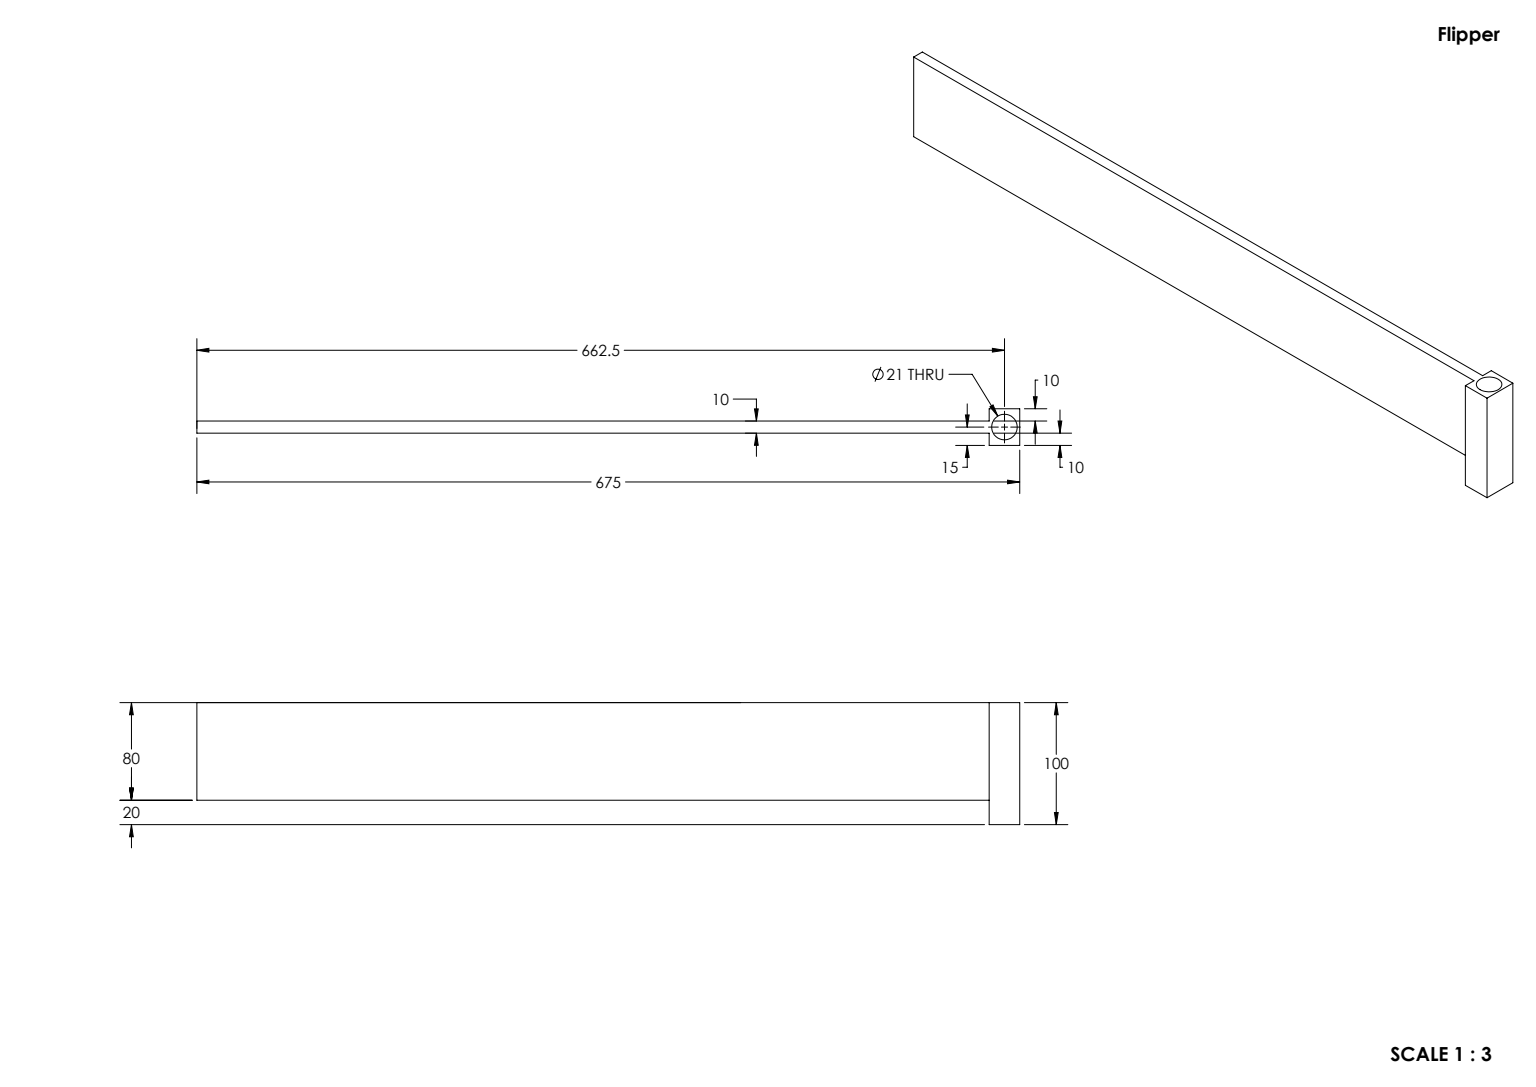
ISO-10303-21;
HEADER;
FILE_DESCRIPTION (('STEP AP214'),
    '1' );
FILE_NAME ('Flipper.step',
    '2026-10-24T15:53:57',
    ( '' ),
    ( '' ),
    'SwSTEP 2.0',
    'SolidWorks 2025',
    '' );
FILE_SCHEMA (( 'AUTOMOTIVE_DESIGN' ));
ENDSEC;

DATA;
#20=MANIFOLD_SOLID_BREP ( 'Cut-Extrude1', #1796 ) ;
#27=EDGE_CURVE ( 'NONE', #6851, #3192, #686, .T. ) ;
#51=PLANE ( 'NONE',  #3089 ) ;
#86=CARTESIAN_POINT ( 'NONE',  ( 5.000000000000115463, -14.99999999999990230, 79.99999999999995737 ) ) ;
#119=CARTESIAN_POINT ( 'NONE',  ( 5.000000000000115463, -14.99999999999990230, 79.99999999999995737 ) ) ;
#159=ORIENTED_EDGE ( 'NONE', *, *, #1330, .T. ) ;
#182=CARTESIAN_POINT ( 'NONE',  ( 10.00000000000012079, -29.14213562373080180, 0.000000000000000000 ) ) ;
#214=ORIENTED_EDGE ( 'NONE', *, *, #1634, .F. ) ;
#218=VERTEX_POINT ( 'NONE', #2995 ) ;
#231=CARTESIAN_POINT ( 'NONE',  ( 5.000000000000115463, -14.99999999999990230, -20.00100000000004741 ) ) ;
#242=VECTOR ( 'NONE', #7821, 1000.000000000000000 ) ;
#252=DIRECTION ( 'NONE',  ( -7.420547859534711256E-34, 1.000000000000000000, 1.224646799147352961E-16 ) ) ;
#253=DIRECTION ( 'NONE',  ( -7.703719777548943412E-34, 0.000000000000000000, 1.000000000000000000 ) ) ;
#256=DIRECTION ( 'NONE',  ( -7.420547859534711256E-34, 1.000000000000000000, 1.224646799147352961E-16 ) ) ;
#261=DIRECTION ( 'NONE',  ( 0.000000000000000000, -1.000000000000000000, -1.224646799147352714E-16 ) ) ;
#262=ADVANCED_FACE ( 'NONE', ( #7614 ), #6970, .T. ) ;
#284=ORIENTED_EDGE ( 'NONE', *, *, #3202, .F. ) ;
#302=ORIENTED_EDGE ( 'NONE', *, *, #1070, .T. ) ;
#303=VERTEX_POINT ( 'NONE', #1894 ) ;
#313=CARTESIAN_POINT ( 'NONE',  ( -9.999999999999884537, -14.99999999999990052, -20.00000000000001776 ) ) ;
#318=ADVANCED_FACE ( 'NONE', ( #509 ), #5075, .F. ) ;
#332=ADVANCED_FACE ( 'NONE', ( #3201 ), #4425, .F. ) ;
#340=CARTESIAN_POINT ( 'NONE',  ( 5.000000000000115463, -14.99999999999990230, -20.00000000000001776 ) ) ;
#359=VECTOR ( 'NONE', #6067, 1000.000000000000000 ) ;
#368=CYLINDRICAL_SURFACE ( 'NONE', #7232, 10.49999999999999645 ) ;
#421=CARTESIAN_POINT ( 'NONE',  ( 9.999999999999896971, 0.000000000000000000, 0.000000000000000000 ) ) ;
#441=CARTESIAN_POINT ( 'NONE',  ( 10.00000000000000888, -650.0000000000002274, 79.99999999999995737 ) ) ;
#458=CARTESIAN_POINT ( 'NONE',  ( 10.00000000000000888, -0.8578643762688908936, 0.000000000000000000 ) ) ;
#479=AXIS2_PLACEMENT_3D ( 'NONE', #3533, #253, #2914 ) ;
#499=DIRECTION ( 'NONE',  ( -7.703719777548943412E-34, 0.000000000000000000, 1.000000000000000000 ) ) ;
#509=FACE_OUTER_BOUND ( 'NONE', #3864, .T. ) ;
#519=ORIENTED_EDGE ( 'NONE', *, *, #7936, .T. ) ;
#530=VERTEX_POINT ( 'NONE', #3474 ) ;
#550=LINE ( 'NONE', #5350, #242 ) ;
#558=EDGE_CURVE ( 'NONE', #4476, #8418, #2901, .T. ) ;
#565=LINE ( 'NONE', #5367, #5443 ) ;
#581=CIRCLE ( 'NONE', #5462, 15.00000000000000355 ) ;
#622=CARTESIAN_POINT ( 'NONE',  ( 5.000000000000004441, 0.000000000000000000, 0.000000000000000000 ) ) ;
#624=ORIENTED_EDGE ( 'NONE', *, *, #8030, .T. ) ;
#627=ORIENTED_EDGE ( 'NONE', *, *, #1962, .T. ) ;
#630=ORIENTED_EDGE ( 'NONE', *, *, #1968, .T. ) ;
#686=LINE ( 'NONE', #6066, #6271 ) ;
#718=ORIENTED_EDGE ( 'NONE', *, *, #558, .T. ) ;
#731=LINE ( 'NONE', #3391, #359 ) ;
#774=( LENGTH_UNIT ( ) NAMED_UNIT ( * ) SI_UNIT ( .MILLI., .METRE. ) );
#800=DIRECTION ( 'NONE',  ( 1.000000000000000000, 0.000000000000000000, 0.000000000000000000 ) ) ;
#826=CIRCLE ( 'NONE', #1930, 10.49999999999999645 ) ;
#832=ORIENTED_EDGE ( 'NONE', *, *, #6918, .T. ) ;
#843=DIRECTION ( 'NONE',  ( 4.622231866529366732E-33, -1.224646799147352961E-16, 1.000000000000000000 ) ) ;
#846=EDGE_CURVE ( 'NONE', #4479, #218, #4939, .T. ) ;
#860=( NAMED_UNIT ( * ) PLANE_ANGLE_UNIT ( ) SI_UNIT ( $, .RADIAN. ) );
#883=VECTOR ( 'NONE', #4658, 1000.000000000000000 ) ;
#898=FACE_OUTER_BOUND ( 'NONE', #6189, .T. ) ;
#899=EDGE_CURVE ( 'NONE', #7534, #6851, #5991, .T. ) ;
#942=CARTESIAN_POINT ( 'NONE',  ( 10.00000000000000888, -650.0000000000002274, 79.99999999999995737 ) ) ;
#959=CIRCLE ( 'NONE', #5553, 15.00000000000000355 ) ;
#961=CARTESIAN_POINT ( 'NONE',  ( 0.000000000000000000, 0.000000000000000000, 0.000000000000000000 ) ) ;
#968=DIRECTION ( 'NONE',  ( -7.703719777548943412E-34, 0.000000000000000000, 1.000000000000000000 ) ) ;
#992=ORIENTED_EDGE ( 'NONE', *, *, #3308, .F. ) ;
#1006=EDGE_LOOP ( 'NONE', ( #2429, #302, #624, #3207, #7185, #3525, #718, #4684 ) ) ;
#1061=CARTESIAN_POINT ( 'NONE',  ( 15.50000000000011191, -14.99999999999990230, 79.99999999999995737 ) ) ;
#1066=FACE_BOUND ( 'NONE', #7624, .T. ) ;
#1070=EDGE_CURVE ( 'NONE', #8094, #5152, #5051, .T. ) ;
#1087=CARTESIAN_POINT ( 'NONE',  ( 5.000000000000115463, -14.99999999999990230, 0.000000000000000000 ) ) ;
#1127=DIRECTION ( 'NONE',  ( 2.842664852890546338E-35, -1.000000000000000000, 0.000000000000000000 ) ) ;
#1132=UNCERTAINTY_MEASURE_WITH_UNIT (LENGTH_MEASURE( 1.000000000000000082E-05 ), #1546, 'distance_accuracy_value', 'NONE');
#1140=AXIS2_PLACEMENT_3D ( 'NONE', #6510, #5843, #8469 ) ;
#1162=ORIENTED_EDGE ( 'NONE', *, *, #899, .F. ) ;
#1170=ADVANCED_FACE ( 'NONE', ( #3127 ), #3214, .F. ) ;
#1253=VECTOR ( 'NONE', #5699, 1000.000000000000000 ) ;
#1255=FACE_OUTER_BOUND ( 'NONE', #4456, .T. ) ;
#1308=CARTESIAN_POINT ( 'NONE',  ( -2.220446049250313081E-13, -650.0000000000000000, -1.110223024625156540E-13 ) ) ;
#1330=EDGE_CURVE ( 'NONE', #530, #3192, #731, .T. ) ;
#1337=VERTEX_POINT ( 'NONE', #8226 ) ;
#1352=CARTESIAN_POINT ( 'NONE',  ( 20.00000000000011369, -14.99999999999990230, 79.99999999999995737 ) ) ;
#1359=ORIENTED_EDGE ( 'NONE', *, *, #3242, .T. ) ;
#1364=CARTESIAN_POINT ( 'NONE',  ( 5.000000000000115463, -14.99999999999990230, 79.99999999999995737 ) ) ;
#1388=LINE ( 'NONE', #5356, #4852 ) ;
#1390=CARTESIAN_POINT ( 'NONE',  ( 15.50000000000011191, -14.99999999999990230, -20.00100000000004741 ) ) ;
#1392=( GEOMETRIC_REPRESENTATION_CONTEXT ( 3 ) GLOBAL_UNCERTAINTY_ASSIGNED_CONTEXT ( ( #7343 ) ) GLOBAL_UNIT_ASSIGNED_CONTEXT ( ( #774, #7439, #8135 ) ) REPRESENTATION_CONTEXT ( 'NONE', 'WORKASPACE' ) );
#1393=DIRECTION ( 'NONE',  ( -1.000000000000000000, 2.842664852890546338E-35, 1.540743955509788340E-33 ) ) ;
#1397=CARTESIAN_POINT ( 'NONE',  ( 5.000000000000115463, -14.99999999999990230, -20.00100000000004741 ) ) ;
#1427=AXIS2_PLACEMENT_3D ( 'NONE', #5540, #6844, #1518 ) ;
#1449=CARTESIAN_POINT ( 'NONE',  ( 9.999999999999896971, 0.000000000000000000, 0.000000000000000000 ) ) ;
#1461=EDGE_CURVE ( 'NONE', #7908, #6954, #5531, .T. ) ;
#1465=DIRECTION ( 'NONE',  ( -1.000000000000000000, 2.842664852890546338E-35, -7.703719777548943412E-34 ) ) ;
#1478=ORIENTED_EDGE ( 'NONE', *, *, #1070, .F. ) ;
#1495=ORIENTED_EDGE ( 'NONE', *, *, #1461, .T. ) ;
#1518=DIRECTION ( 'NONE',  ( 1.000000000000000000, 0.000000000000000000, 0.000000000000000000 ) ) ;
#1546=( LENGTH_UNIT ( ) NAMED_UNIT ( * ) SI_UNIT ( .MILLI., .METRE. ) );
#1549=ORIENTED_EDGE ( 'NONE', *, *, #4424, .T. ) ;
#1552=CARTESIAN_POINT ( 'NONE',  ( 0.000000000000000000, 0.000000000000000000, 0.000000000000000000 ) ) ;
#1582=CARTESIAN_POINT ( 'NONE',  ( 9.999999999999896971, 0.000000000000000000, 79.99999999999995737 ) ) ;
#1584=EDGE_CURVE ( 'NONE', #8094, #2182, #6432, .T. ) ;
#1620=DIRECTION ( 'NONE',  ( -1.000000000000000000, 2.842664852890546338E-35, 1.540743955509788340E-33 ) ) ;
#1634=EDGE_CURVE ( 'NONE', #2098, #1337, #5074, .T. ) ;
#1646=CARTESIAN_POINT ( 'NONE',  ( 5.000000000000115463, -14.99999999999990230, 0.000000000000000000 ) ) ;
#1660=AXIS2_PLACEMENT_3D ( 'NONE', #1364, #4015, #6635 ) ;
#1661=EDGE_CURVE ( 'NONE', #1337, #4479, #4550, .T. ) ;
#1716=VERTEX_POINT ( 'NONE', #3373 ) ;
#1748=VECTOR ( 'NONE', #8434, 1000.000000000000000 ) ;
#1757=ORIENTED_EDGE ( 'NONE', *, *, #1584, .T. ) ;
#1766=ADVANCED_FACE ( 'NONE', ( #6825 ), #2170, .T. ) ;
#1775=CARTESIAN_POINT ( 'NONE',  ( 5.000000000000115463, -14.99999999999990230, -20.00000000000001776 ) ) ;
#1796=CLOSED_SHELL ( 'NONE', ( #5165, #5744, #3088, #4851, #318, #262, #4059, #4277, #1170, #4627, #332, #5630, #1766, #4762, #3103 ) ) ;
#1823=DIRECTION ( 'NONE',  ( 1.000000000000000000, -2.842664852890546338E-35, -1.540743955509788340E-33 ) ) ;
#1835=AXIS2_PLACEMENT_3D ( 'NONE', #1397, #4571, #7970 ) ;
#1838=ORIENTED_EDGE ( 'NONE', *, *, #6705, .F. ) ;
#1894=CARTESIAN_POINT ( 'NONE',  ( 0.000000000000000000, 0.000000000000000000, 79.99999999999995737 ) ) ;
#1908=DIRECTION ( 'NONE',  ( -2.842664852890546338E-35, 1.000000000000000000, -2.189909344815615958E-68 ) ) ;
#1918=CARTESIAN_POINT ( 'NONE',  ( 9.999999999999896971, 0.000000000000000000, 0.000000000000000000 ) ) ;
#1930=AXIS2_PLACEMENT_3D ( 'NONE', #3172, #8488, #2522 ) ;
#1935=EDGE_LOOP ( 'NONE', ( #6404, #7360, #7630 ) ) ;
#1962=EDGE_CURVE ( 'NONE', #2182, #8418, #8061, .T. ) ;
#1968=EDGE_CURVE ( 'NONE', #5323, #2931, #2361, .T. ) ;
#2048=ORIENTED_EDGE ( 'NONE', *, *, #5752, .F. ) ;
#2098=VERTEX_POINT ( 'NONE', #458 ) ;
#2105=AXIS2_PLACEMENT_3D ( 'NONE', #1646, #2967, #261 ) ;
#2128=FACE_OUTER_BOUND ( 'NONE', #4821, .T. ) ;
#2132=EDGE_CURVE ( 'NONE', #8150, #6642, #5440, .T. ) ;
#2157=APPLICATION_CONTEXT ( 'automotive_design' ) ;
#2170=CYLINDRICAL_SURFACE ( 'NONE', #3581, 15.00000000000000355 ) ;
#2178=EDGE_CURVE ( 'NONE', #218, #303, #4541, .T. ) ;
#2182=VERTEX_POINT ( 'NONE', #7938 ) ;
#2248=EDGE_LOOP ( 'NONE', ( #6424, #4523 ) ) ;
#2261=AXIS2_PLACEMENT_3D ( 'NONE', #7188, #5267, #6624 ) ;
#2279=DIRECTION ( 'NONE',  ( 1.000000000000000000, 0.000000000000000000, 0.000000000000000000 ) ) ;
#2306=VECTOR ( 'NONE', #2824, 1000.000000000000000 ) ;
#2357=VECTOR ( 'NONE', #7940, 1000.000000000000000 ) ;
#2361=LINE ( 'NONE', #7639, #2490 ) ;
#2370=CIRCLE ( 'NONE', #4607, 10.49999999999999645 ) ;
#2416=DIRECTION ( 'NONE',  ( 2.842664852890546338E-35, -1.000000000000000000, 0.000000000000000000 ) ) ;
#2429=ORIENTED_EDGE ( 'NONE', *, *, #1584, .F. ) ;
#2440=CARTESIAN_POINT ( 'NONE',  ( 9.999999999999896971, 0.000000000000000000, 79.99999999999995737 ) ) ;
#2442=ORIENTED_EDGE ( 'NONE', *, *, #1634, .T. ) ;
#2470=CARTESIAN_POINT ( 'NONE',  ( 15.50000000000011191, -14.99999999999990230, -20.00000000000001776 ) ) ;
#2477=AXIS2_PLACEMENT_3D ( 'NONE', #1775, #7223, #3788 ) ;
#2490=VECTOR ( 'NONE', #3020, 1000.000000000000000 ) ;
#2522=DIRECTION ( 'NONE',  ( 1.000000000000000000, 0.000000000000000000, 0.000000000000000000 ) ) ;
#2533=CIRCLE ( 'NONE', #1427, 10.49999999999999645 ) ;
#2542=VECTOR ( 'NONE', #4532, 1000.000000000000000 ) ;
#2613=CARTESIAN_POINT ( 'NONE',  ( 10.00000000000000888, -650.0000000000002274, 79.99999999999995737 ) ) ;
#2654=CARTESIAN_POINT ( 'NONE',  ( -2.220446049250313081E-13, -650.0000000000000000, 79.99999999999995737 ) ) ;
#2704=EDGE_CURVE ( 'NONE', #1716, #303, #6156, .T. ) ;
#2707=ORIENTED_EDGE ( 'NONE', *, *, #6829, .T. ) ;
#2759=AXIS2_PLACEMENT_3D ( 'NONE', #6982, #3002, #8237 ) ;
#2824=DIRECTION ( 'NONE',  ( -7.703719777548943412E-34, 0.000000000000000000, 1.000000000000000000 ) ) ;
#2837=EDGE_LOOP ( 'NONE', ( #1359, #5314, #2707, #5174 ) ) ;
#2852=ORIENTED_EDGE ( 'NONE', *, *, #6705, .T. ) ;
#2874=ORIENTED_EDGE ( 'NONE', *, *, #5062, .T. ) ;
#2901=LINE ( 'NONE', #7568, #8115 ) ;
#2914=DIRECTION ( 'NONE',  ( 1.000000000000000000, 0.000000000000000000, 0.000000000000000000 ) ) ;
#2917=CARTESIAN_POINT ( 'NONE',  ( 10.00000000000000888, -0.8578643762688908936, -20.00000000000001776 ) ) ;
#2931=VERTEX_POINT ( 'NONE', #4996 ) ;
#2967=DIRECTION ( 'NONE',  ( 4.622231866529366047E-33, -1.224646799147353454E-16, 1.000000000000000000 ) ) ;
#2987=EDGE_CURVE ( 'NONE', #3472, #6642, #8000, .T. ) ;
#2995=CARTESIAN_POINT ( 'NONE',  ( 0.000000000000000000, 0.000000000000000000, 0.000000000000000000 ) ) ;
#3002=DIRECTION ( 'NONE',  ( -7.703719777548943412E-34, 0.000000000000000000, 1.000000000000000000 ) ) ;
#3013=VECTOR ( 'NONE', #5841, 1000.000000000000000 ) ;
#3020=DIRECTION ( 'NONE',  ( 7.703719777548943412E-34, -0.000000000000000000, -1.000000000000000000 ) ) ;
#3030=APPLICATION_CONTEXT ( 'automotive_design' ) ;
#3070=LINE ( 'NONE', #421, #6723 ) ;
#3078=CARTESIAN_POINT ( 'NONE',  ( 0.000000000000000000, -29.14213562373091548, 79.99999999999995737 ) ) ;
#3079=EDGE_LOOP ( 'NONE', ( #2852, #1757, #6501, #630, #284, #2048, #8486, #7214, #4382 ) ) ;
#3088=ADVANCED_FACE ( 'NONE', ( #3867 ), #4666, .F. ) ;
#3089=AXIS2_PLACEMENT_3D ( 'NONE', #1582, #4894, #8083 ) ;
#3103=ADVANCED_FACE ( 'NONE', ( #1255 ), #3351, .F. ) ;
#3127=FACE_OUTER_BOUND ( 'NONE', #6595, .T. ) ;
#3141=CARTESIAN_POINT ( 'NONE',  ( 20.00000000000011724, -14.99999999999990230, -20.00000000000001776 ) ) ;
#3144=ADVANCED_BREP_SHAPE_REPRESENTATION ( '', ( #20, #7563 ), #4918 ) ;
#3152=ORIENTED_EDGE ( 'NONE', *, *, #2132, .F. ) ;
#3159=AXIS2_PLACEMENT_3D ( 'NONE', #1918, #4576, #7231 ) ;
#3172=CARTESIAN_POINT ( 'NONE',  ( 5.000000000000115463, -14.99999999999990230, 79.99999999999995737 ) ) ;
#3192=VERTEX_POINT ( 'NONE', #1308 ) ;
#3201=FACE_OUTER_BOUND ( 'NONE', #5224, .T. ) ;
#3202=EDGE_CURVE ( 'NONE', #4479, #2931, #581, .T. ) ;
#3207=ORIENTED_EDGE ( 'NONE', *, *, #7936, .F. ) ;
#3214=PLANE ( 'NONE',  #4107 ) ;
#3220=ORIENTED_EDGE ( 'NONE', *, *, #2132, .T. ) ;
#3242=EDGE_CURVE ( 'NONE', #6699, #3472, #2533, .T. ) ;
#3271=PRODUCT ( 'Flipper', 'Flipper', '', ( #5996 ) ) ;
#3275=CARTESIAN_POINT ( 'NONE',  ( 10.00000000000000888, -650.0000000000002274, -1.110223024625156540E-13 ) ) ;
#3306=DIRECTION ( 'NONE',  ( -7.703719777548943412E-34, 0.000000000000000000, 1.000000000000000000 ) ) ;
#3308=EDGE_CURVE ( 'NONE', #530, #7908, #3070, .T. ) ;
#3351=CYLINDRICAL_SURFACE ( 'NONE', #1835, 10.49999999999999645 ) ;
#3355=EDGE_LOOP ( 'NONE', ( #1838, #1478 ) ) ;
#3358=SHAPE_DEFINITION_REPRESENTATION ( #7238, #6122 ) ;
#3373=CARTESIAN_POINT ( 'NONE',  ( 9.999999999999896971, 0.000000000000000000, 79.99999999999995737 ) ) ;
#3375=VECTOR ( 'NONE', #7753, 1000.000000000000000 ) ;
#3391=CARTESIAN_POINT ( 'NONE',  ( 10.00000000000000888, -650.0000000000002274, -1.110223024625156540E-13 ) ) ;
#3408=PRODUCT_DEFINITION_FORMATION_WITH_SPECIFIED_SOURCE ( 'ANY', '', #3271, .NOT_KNOWN. ) ;
#3420=EDGE_CURVE ( 'NONE', #8418, #6851, #3888, .T. ) ;
#3423=CARTESIAN_POINT ( 'NONE',  ( 5.000000000000115463, -14.99999999999990230, -20.00000000000001776 ) ) ;
#3445=DIRECTION ( 'NONE',  ( 0.000000000000000000, -1.000000000000000000, -1.224646799147352714E-16 ) ) ;
#3457=VECTOR ( 'NONE', #256, 1000.000000000000000 ) ;
#3472=VERTEX_POINT ( 'NONE', #7162 ) ;
#3474=CARTESIAN_POINT ( 'NONE',  ( 10.00000000000000888, -650.0000000000002274, -1.110223024625156540E-13 ) ) ;
#3478=LINE ( 'NONE', #1390, #4927 ) ;
#3485=CARTESIAN_POINT ( 'NONE',  ( 5.000000000000115463, -14.99999999999990230, 0.000000000000000000 ) ) ;
#3512=DIRECTION ( 'NONE',  ( 1.000000000000000000, 0.000000000000000000, 0.000000000000000000 ) ) ;
#3525=ORIENTED_EDGE ( 'NONE', *, *, #6695, .F. ) ;
#3533=CARTESIAN_POINT ( 'NONE',  ( 5.000000000000115463, -14.99999999999990230, -20.00000000000001776 ) ) ;
#3581=AXIS2_PLACEMENT_3D ( 'NONE', #3423, #8256, #6787 ) ;
#3589=CARTESIAN_POINT ( 'NONE',  ( 5.000000000000115463, -14.99999999999990230, -20.00000000000001776 ) ) ;
#3592=ORIENTED_EDGE ( 'NONE', *, *, #2704, .F. ) ;
#3621=DIRECTION ( 'NONE',  ( 7.703719777548943412E-34, -0.000000000000000000, -1.000000000000000000 ) ) ;
#3640=DIRECTION ( 'NONE',  ( -7.703719777548943412E-34, 0.000000000000000000, 1.000000000000000000 ) ) ;
#3643=DIRECTION ( 'NONE',  ( -1.540743955509788340E-33, 6.569728034446847052E-68, -1.000000000000000000 ) ) ;
#3649=ORIENTED_EDGE ( 'NONE', *, *, #3308, .T. ) ;
#3712=CARTESIAN_POINT ( 'NONE',  ( 2.220446049250313081E-13, -0.8578643762688908936, 79.99999999999995737 ) ) ;
#3718=ORIENTED_EDGE ( 'NONE', *, *, #2987, .F. ) ;
#3759=AXIS2_PLACEMENT_3D ( 'NONE', #86, #4811, #800 ) ;
#3788=DIRECTION ( 'NONE',  ( 1.000000000000000000, 0.000000000000000000, 0.000000000000000000 ) ) ;
#3790=EDGE_LOOP ( 'NONE', ( #8491, #519, #1549, #7462, #5645, #832, #4157, #627, #5413, #1162 ) ) ;
#3857=ORIENTED_EDGE ( 'NONE', *, *, #1330, .F. ) ;
#3862=ORIENTED_EDGE ( 'NONE', *, *, #2178, .T. ) ;
#3864=EDGE_LOOP ( 'NONE', ( #3649, #1495, #2874, #6155 ) ) ;
#3867=FACE_OUTER_BOUND ( 'NONE', #6354, .T. ) ;
#3871=VECTOR ( 'NONE', #5283, 1000.000000000000000 ) ;
#3883=STYLED_ITEM('',(#8677),#20);
#3888=LINE ( 'NONE', #8385, #5627 ) ;
#3894=CARTESIAN_POINT ( 'NONE',  ( 9.999999999999896971, 0.000000000000000000, 0.000000000000000000 ) ) ;
#3914=PLANE ( 'NONE',  #6054 ) ;
#4015=DIRECTION ( 'NONE',  ( -7.703719777548943412E-34, 0.000000000000000000, 1.000000000000000000 ) ) ;
#4059=ADVANCED_FACE ( 'NONE', ( #898 ), #51, .F. ) ;
#4105=DIRECTION ( 'NONE',  ( 7.420547859534711256E-34, -1.000000000000000000, -1.224646799147352961E-16 ) ) ;
#4107=AXIS2_PLACEMENT_3D ( 'NONE', #5898, #1908, #4520 ) ;
#4126=DIRECTION ( 'NONE',  ( 7.703719777548943412E-34, 0.000000000000000000, -1.000000000000000000 ) ) ;
#4144=CIRCLE ( 'NONE', #2759, 15.00000000000000355 ) ;
#4153=ORIENTED_EDGE ( 'NONE', *, *, #7725, .F. ) ;
#4157=ORIENTED_EDGE ( 'NONE', *, *, #6583, .T. ) ;
#4203=CARTESIAN_POINT ( 'NONE',  ( 0.000000000000000000, 0.000000000000000000, 0.000000000000000000 ) ) ;
#4277=ADVANCED_FACE ( 'NONE', ( #1066, #8254 ), #6306, .F. ) ;
#4285=CARTESIAN_POINT ( 'NONE',  ( 9.999999999999896971, 0.000000000000000000, 0.000000000000000000 ) ) ;
#4290=PRODUCT_DEFINITION ( 'UNKNOWN', '', #3408, #6551 ) ;
#4335=CARTESIAN_POINT ( 'NONE',  ( 5.000000000000115463, -14.99999999999990230, 79.99999999999995737 ) ) ;
#4382=ORIENTED_EDGE ( 'NONE', *, *, #8030, .F. ) ;
#4400=DIRECTION ( 'NONE',  ( 4.622231866529366047E-33, -1.224646799147353454E-16, 1.000000000000000000 ) ) ;
#4408=ORIENTED_EDGE ( 'NONE', *, *, #899, .T. ) ;
#4424=EDGE_CURVE ( 'NONE', #4437, #6290, #5319, .T. ) ;
#4425=PLANE ( 'NONE',  #7545 ) ;
#4437=VERTEX_POINT ( 'NONE', #1352 ) ;
#4453=AXIS2_PLACEMENT_3D ( 'NONE', #3589, #968, #6250 ) ;
#4456=EDGE_LOOP ( 'NONE', ( #3718, #8082, #8564, #3220 ) ) ;
#4465=DIRECTION ( 'NONE',  ( -7.703719777548943412E-34, 0.000000000000000000, 1.000000000000000000 ) ) ;
#4476=VERTEX_POINT ( 'NONE', #7935 ) ;
#4479=VERTEX_POINT ( 'NONE', #622 ) ;
#4482=FACE_BOUND ( 'NONE', #2248, .T. ) ;
#4517=ORIENTED_EDGE ( 'NONE', *, *, #2178, .F. ) ;
#4520=DIRECTION ( 'NONE',  ( -7.703719777548943412E-34, 0.000000000000000000, 1.000000000000000000 ) ) ;
#4523=ORIENTED_EDGE ( 'NONE', *, *, #5859, .F. ) ;
#4531=FACE_OUTER_BOUND ( 'NONE', #1935, .T. ) ;
#4532=DIRECTION ( 'NONE',  ( -1.000000000000000000, 2.842664852890546338E-35, 1.540743955509788340E-33 ) ) ;
#4541=LINE ( 'NONE', #7199, #3871 ) ;
#4546=DIRECTION ( 'NONE',  ( -7.420547859534711256E-34, 1.000000000000000000, 1.224646799147352961E-16 ) ) ;
#4550=LINE ( 'NONE', #3894, #7883 ) ;
#4571=DIRECTION ( 'NONE',  ( -7.703719777548943412E-34, 0.000000000000000000, 1.000000000000000000 ) ) ;
#4576=DIRECTION ( 'NONE',  ( 4.622231866529366732E-33, -1.224646799147352961E-16, 1.000000000000000000 ) ) ;
#4607=AXIS2_PLACEMENT_3D ( 'NONE', #340, #7653, #8310 ) ;
#4620=ORIENTED_EDGE ( 'NONE', *, *, #1968, .F. ) ;
#4627=ADVANCED_FACE ( 'NONE', ( #7416 ), #6815, .F. ) ;
#4658=DIRECTION ( 'NONE',  ( -1.000000000000000000, 2.842664852890546338E-35, 1.540743955509788340E-33 ) ) ;
#4666=PLANE ( 'NONE',  #2261 ) ;
#4684=ORIENTED_EDGE ( 'NONE', *, *, #1962, .F. ) ;
#4750=DIRECTION ( 'NONE',  ( -7.703719777548943412E-34, 0.000000000000000000, 1.000000000000000000 ) ) ;
#4762=ADVANCED_FACE ( 'NONE', ( #4482, #6628 ), #3914, .F. ) ;
#4781=PLANE ( 'NONE',  #5088 ) ;
#4788=CARTESIAN_POINT ( 'NONE',  ( 10.00000000000012079, -29.14213562373080180, -20.00000000000001776 ) ) ;
#4811=DIRECTION ( 'NONE',  ( -7.703719777548943412E-34, 0.000000000000000000, 1.000000000000000000 ) ) ;
#4821=EDGE_LOOP ( 'NONE', ( #4620, #6513, #4517, #5324 ) ) ;
#4836=LINE ( 'NONE', #961, #3457 ) ;
#4851=ADVANCED_FACE ( 'NONE', ( #4531 ), #7190, .F. ) ;
#4852=VECTOR ( 'NONE', #7349, 1000.000000000000000 ) ;
#4856=ORIENTED_EDGE ( 'NONE', *, *, #6794, .T. ) ;
#4892=CARTESIAN_POINT ( 'NONE',  ( 20.00000000000011724, -14.99999999999990230, -20.00000000000001776 ) ) ;
#4894=DIRECTION ( 'NONE',  ( 2.960372000631175920E-34, -1.000000000000000000, -4.592425496802573602E-17 ) ) ;
#4918=( GEOMETRIC_REPRESENTATION_CONTEXT ( 3 ) GLOBAL_UNCERTAINTY_ASSIGNED_CONTEXT ( ( #1132 ) ) GLOBAL_UNIT_ASSIGNED_CONTEXT ( ( #1546, #860, #7644 ) ) REPRESENTATION_CONTEXT ( 'NONE', 'WORKASPACE' ) );
#4927=VECTOR ( 'NONE', #4750, 1000.000000000000000 ) ;
#4934=ORIENTED_EDGE ( 'NONE', *, *, #6341, .T. ) ;
#4937=CARTESIAN_POINT ( 'NONE',  ( 10.00000000000000888, -650.0000000000002274, 79.99999999999995737 ) ) ;
#4939=LINE ( 'NONE', #4285, #2542 ) ;
#4984=ORIENTED_EDGE ( 'NONE', *, *, #27, .T. ) ;
#4986=CIRCLE ( 'NONE', #2477, 15.00000000000000355 ) ;
#4996=CARTESIAN_POINT ( 'NONE',  ( 2.220446049250313081E-13, -0.8578643762688908936, -1.110223024625156540E-13 ) ) ;
#5051=CIRCLE ( 'NONE', #479, 15.00000000000000355 ) ;
#5062=EDGE_CURVE ( 'NONE', #6954, #7534, #550, .T. ) ;
#5074=LINE ( 'NONE', #7729, #3013 ) ;
#5075=PLANE ( 'NONE',  #1140 ) ;
#5088=AXIS2_PLACEMENT_3D ( 'NONE', #7434, #1465, #6145 ) ;
#5152=VERTEX_POINT ( 'NONE', #4892 ) ;
#5165=ADVANCED_FACE ( 'NONE', ( #8251 ), #368, .F. ) ;
#5174=ORIENTED_EDGE ( 'NONE', *, *, #8192, .F. ) ;
#5193=VECTOR ( 'NONE', #6792, 1000.000000000000000 ) ;
#5224=EDGE_LOOP ( 'NONE', ( #4856, #5475, #2442, #4934 ) ) ;
#5254=ORIENTED_EDGE ( 'NONE', *, *, #846, .T. ) ;
#5267=DIRECTION ( 'NONE',  ( 4.622231866529366732E-33, -1.224646799147352961E-16, 1.000000000000000000 ) ) ;
#5283=DIRECTION ( 'NONE',  ( -1.540743955509788682E-33, -4.592425496802573602E-17, 1.000000000000000000 ) ) ;
#5286=CIRCLE ( 'NONE', #2105, 15.00000000000000355 ) ;
#5314=ORIENTED_EDGE ( 'NONE', *, *, #2987, .T. ) ;
#5319=CIRCLE ( 'NONE', #5326, 15.00000000000000355 ) ;
#5323=VERTEX_POINT ( 'NONE', #3712 ) ;
#5324=ORIENTED_EDGE ( 'NONE', *, *, #6612, .F. ) ;
#5326=AXIS2_PLACEMENT_3D ( 'NONE', #119, #3306, #7403 ) ;
#5331=AXIS2_PLACEMENT_3D ( 'NONE', #4937, #3643, #1620 ) ;
#5350=CARTESIAN_POINT ( 'NONE',  ( 10.00000000000000888, -650.0000000000002274, 79.99999999999995737 ) ) ;
#5356=CARTESIAN_POINT ( 'NONE',  ( -2.220446049250313081E-13, -650.0000000000000000, 79.99999999999995737 ) ) ;
#5367=CARTESIAN_POINT ( 'NONE',  ( 0.000000000000000000, 0.000000000000000000, 0.000000000000000000 ) ) ;
#5413=ORIENTED_EDGE ( 'NONE', *, *, #3420, .T. ) ;
#5425=ORIENTED_EDGE ( 'NONE', *, *, #27, .F. ) ;
#5440=CIRCLE ( 'NONE', #1660, 10.49999999999999645 ) ;
#5443=VECTOR ( 'NONE', #252, 1000.000000000000000 ) ;
#5462=AXIS2_PLACEMENT_3D ( 'NONE', #3485, #5497, #3445 ) ;
#5475=ORIENTED_EDGE ( 'NONE', *, *, #6627, .T. ) ;
#5480=ORIENTED_EDGE ( 'NONE', *, *, #5789, .T. ) ;
#5497=DIRECTION ( 'NONE',  ( 4.622231866529366047E-33, -1.224646799147353454E-16, 1.000000000000000000 ) ) ;
#5531=LINE ( 'NONE', #4788, #2306 ) ;
#5536=ORIENTED_EDGE ( 'NONE', *, *, #1661, .F. ) ;
#5540=CARTESIAN_POINT ( 'NONE',  ( 5.000000000000115463, -14.99999999999990230, -20.00000000000001776 ) ) ;
#5553=AXIS2_PLACEMENT_3D ( 'NONE', #1087, #4400, #5901 ) ;
#5568=SHAPE_REPRESENTATION_RELATIONSHIP ( 'NONE' , 'NONE' ,  #6122, #3144 ) ;
#5627=VECTOR ( 'NONE', #2416, 1000.000000000000000 ) ;
#5630=ADVANCED_FACE ( 'NONE', ( #2128 ), #4781, .T. ) ;
#5644=LINE ( 'NONE', #2917, #6384 ) ;
#5645=ORIENTED_EDGE ( 'NONE', *, *, #2704, .T. ) ;
#5676=DIRECTION ( 'NONE',  ( -7.703719777548943412E-34, 0.000000000000000000, 1.000000000000000000 ) ) ;
#5699=DIRECTION ( 'NONE',  ( -7.703719777548943412E-34, 0.000000000000000000, 1.000000000000000000 ) ) ;
#5744=ADVANCED_FACE ( 'NONE', ( #7543 ), #8195, .T. ) ;
#5750=ORIENTED_EDGE ( 'NONE', *, *, #1661, .T. ) ;
#5752=EDGE_CURVE ( 'NONE', #2098, #4479, #5286, .T. ) ;
#5789=EDGE_CURVE ( 'NONE', #3192, #4476, #565, .T. ) ;
#5827=LINE ( 'NONE', #3141, #1253 ) ;
#5841=DIRECTION ( 'NONE',  ( -7.420547859534711256E-34, 1.000000000000000000, 1.224646799147352961E-16 ) ) ;
#5843=DIRECTION ( 'NONE',  ( -1.000000000000000000, 2.842664852890546338E-35, -7.703719777548943412E-34 ) ) ;
#5859=EDGE_CURVE ( 'NONE', #3472, #6699, #2370, .T. ) ;
#5898=CARTESIAN_POINT ( 'NONE',  ( 10.00000000000000888, -650.0000000000002274, -1.110223024625156540E-13 ) ) ;
#5901=DIRECTION ( 'NONE',  ( 0.000000000000000000, -1.000000000000000000, -1.224646799147352714E-16 ) ) ;
#5990=DIRECTION ( 'NONE',  ( 1.540743955509788340E-33, -6.569728034446847052E-68, 1.000000000000000000 ) ) ;
#5991=LINE ( 'NONE', #2613, #883 ) ;
#5996=PRODUCT_CONTEXT ( 'NONE', #2157, 'mechanical' ) ;
#6054=AXIS2_PLACEMENT_3D ( 'NONE', #6532, #5990, #1823 ) ;
#6066=CARTESIAN_POINT ( 'NONE',  ( -2.220446049250313081E-13, -650.0000000000000000, -1.110223024625156540E-13 ) ) ;
#6067=DIRECTION ( 'NONE',  ( -1.000000000000000000, 2.842664852890546338E-35, 1.540743955509788340E-33 ) ) ;
#6120=ORIENTED_EDGE ( 'NONE', *, *, #6695, .T. ) ;
#6122=SHAPE_REPRESENTATION ( 'Flipper', ( #7563 ), #4918 ) ;
#6129=VECTOR ( 'NONE', #1127, 1000.000000000000000 ) ;
#6145=DIRECTION ( 'NONE',  ( -7.703719777548943412E-34, 0.000000000000000000, 1.000000000000000000 ) ) ;
#6148=CIRCLE ( 'NONE', #3759, 15.00000000000000355 ) ;
#6155=ORIENTED_EDGE ( 'NONE', *, *, #7725, .T. ) ;
#6156=LINE ( 'NONE', #6803, #7783 ) ;
#6189=EDGE_LOOP ( 'NONE', ( #5750, #5254, #3862, #3592, #8584 ) ) ;
#6210=ORIENTED_EDGE ( 'NONE', *, *, #6829, .F. ) ;
#6250=DIRECTION ( 'NONE',  ( 1.000000000000000000, 0.000000000000000000, 0.000000000000000000 ) ) ;
#6271=VECTOR ( 'NONE', #4126, 1000.000000000000000 ) ;
#6290=VERTEX_POINT ( 'NONE', #7234 ) ;
#6306=PLANE ( 'NONE',  #5331 ) ;
#6341=EDGE_CURVE ( 'NONE', #1337, #1716, #8416, .T. ) ;
#6354=EDGE_LOOP ( 'NONE', ( #214, #8221, #5536 ) ) ;
#6361=CARTESIAN_POINT ( 'NONE',  ( -9.999999999999888090, -14.99999999999990052, -20.00000000000001776 ) ) ;
#6384=VECTOR ( 'NONE', #3621, 1000.000000000000000 ) ;
#6404=ORIENTED_EDGE ( 'NONE', *, *, #846, .F. ) ;
#6424=ORIENTED_EDGE ( 'NONE', *, *, #3242, .F. ) ;
#6432=LINE ( 'NONE', #6361, #1748 ) ;
#6461=DIRECTION ( 'NONE',  ( 1.000000000000000000, 0.000000000000000000, 0.000000000000000000 ) ) ;
#6476=ORIENTED_EDGE ( 'NONE', *, *, #558, .F. ) ;
#6501=ORIENTED_EDGE ( 'NONE', *, *, #6583, .F. ) ;
#6510=CARTESIAN_POINT ( 'NONE',  ( 9.999999999999896971, 0.000000000000000000, 0.000000000000000000 ) ) ;
#6513=ORIENTED_EDGE ( 'NONE', *, *, #6918, .F. ) ;
#6532=CARTESIAN_POINT ( 'NONE',  ( 5.000000000000115463, -14.99999999999990230, -20.00000000000001776 ) ) ;
#6551=PRODUCT_DEFINITION_CONTEXT ( 'detailed design', #3030, 'design' ) ;
#6583=EDGE_CURVE ( 'NONE', #5323, #2182, #4144, .T. ) ;
#6595=EDGE_LOOP ( 'NONE', ( #4984, #3857, #4153, #4408 ) ) ;
#6612=EDGE_CURVE ( 'NONE', #2931, #218, #4836, .T. ) ;
#6624=DIRECTION ( 'NONE',  ( 7.420547859534711256E-34, -1.000000000000000000, -1.224646799147352961E-16 ) ) ;
#6627=EDGE_CURVE ( 'NONE', #6290, #2098, #5644, .T. ) ;
#6628=FACE_OUTER_BOUND ( 'NONE', #3355, .T. ) ;
#6635=DIRECTION ( 'NONE',  ( 1.000000000000000000, 0.000000000000000000, 0.000000000000000000 ) ) ;
#6642=VERTEX_POINT ( 'NONE', #7581 ) ;
#6678=MECHANICAL_DESIGN_GEOMETRIC_PRESENTATION_REPRESENTATION('',(#3883),#1392);
#6695=EDGE_CURVE ( 'NONE', #4476, #7908, #959, .T. ) ;
#6699=VERTEX_POINT ( 'NONE', #2470 ) ;
#6705=EDGE_CURVE ( 'NONE', #5152, #8094, #4986, .T. ) ;
#6723=VECTOR ( 'NONE', #4546, 1000.000000000000000 ) ;
#6729=LINE ( 'NONE', #3275, #2357 ) ;
#6736=AXIS2_PLACEMENT_3D ( 'NONE', #1449, #843, #4105 ) ;
#6787=DIRECTION ( 'NONE',  ( 1.000000000000000000, 0.000000000000000000, 0.000000000000000000 ) ) ;
#6792=DIRECTION ( 'NONE',  ( -7.703719777548943412E-34, 0.000000000000000000, 1.000000000000000000 ) ) ;
#6794=EDGE_CURVE ( 'NONE', #1716, #6290, #7705, .T. ) ;
#6803=CARTESIAN_POINT ( 'NONE',  ( 9.999999999999896971, 0.000000000000000000, 79.99999999999995737 ) ) ;
#6815=PLANE ( 'NONE',  #6736 ) ;
#6825=FACE_OUTER_BOUND ( 'NONE', #1006, .T. ) ;
#6829=EDGE_CURVE ( 'NONE', #6642, #8150, #826, .T. ) ;
#6838=DIRECTION ( 'NONE',  ( -1.000000000000000000, 2.842664852890546338E-35, -7.703719777548943412E-34 ) ) ;
#6844=DIRECTION ( 'NONE',  ( 7.703719777548943412E-34, -0.000000000000000000, -1.000000000000000000 ) ) ;
#6851=VERTEX_POINT ( 'NONE', #2654 ) ;
#6918=EDGE_CURVE ( 'NONE', #303, #5323, #1388, .T. ) ;
#6954=VERTEX_POINT ( 'NONE', #6972 ) ;
#6970=PLANE ( 'NONE',  #8103 ) ;
#6972=CARTESIAN_POINT ( 'NONE',  ( 10.00000000000012079, -29.14213562373080180, 79.99999999999995737 ) ) ;
#6982=CARTESIAN_POINT ( 'NONE',  ( 5.000000000000115463, -14.99999999999990230, 79.99999999999995737 ) ) ;
#7054=EDGE_LOOP ( 'NONE', ( #5480, #6120, #992, #159 ) ) ;
#7162=CARTESIAN_POINT ( 'NONE',  ( -5.499999999999880096, -14.99999999999990052, -20.00000000000001776 ) ) ;
#7185=ORIENTED_EDGE ( 'NONE', *, *, #1461, .F. ) ;
#7188=CARTESIAN_POINT ( 'NONE',  ( 9.999999999999896971, 0.000000000000000000, 0.000000000000000000 ) ) ;
#7190=PLANE ( 'NONE',  #3159 ) ;
#7199=CARTESIAN_POINT ( 'NONE',  ( 0.000000000000000000, 0.000000000000000000, 79.99999999999995737 ) ) ;
#7200=EDGE_LOOP ( 'NONE', ( #6476, #7592, #5425, #7450 ) ) ;
#7214=ORIENTED_EDGE ( 'NONE', *, *, #4424, .F. ) ;
#7223=DIRECTION ( 'NONE',  ( -7.703719777548943412E-34, 0.000000000000000000, 1.000000000000000000 ) ) ;
#7231=DIRECTION ( 'NONE',  ( 7.420547859534711256E-34, -1.000000000000000000, -1.224646799147352961E-16 ) ) ;
#7232=AXIS2_PLACEMENT_3D ( 'NONE', #231, #3640, #2279 ) ;
#7234=CARTESIAN_POINT ( 'NONE',  ( 10.00000000000000888, -0.8578643762688908936, 79.99999999999995737 ) ) ;
#7238=PRODUCT_DEFINITION_SHAPE ( 'NONE', 'NONE',  #4290 ) ;
#7301=CARTESIAN_POINT ( 'NONE',  ( -5.499999999999881872, -14.99999999999990052, -20.00100000000004741 ) ) ;
#7343=UNCERTAINTY_MEASURE_WITH_UNIT (LENGTH_MEASURE( 1.000000000000000082E-05 ), #774, 'distance_accuracy_value', 'NONE');
#7349=DIRECTION ( 'NONE',  ( 2.842664852890546338E-35, -1.000000000000000000, 0.000000000000000000 ) ) ;
#7360=ORIENTED_EDGE ( 'NONE', *, *, #3202, .T. ) ;
#7403=DIRECTION ( 'NONE',  ( 1.000000000000000000, 0.000000000000000000, 0.000000000000000000 ) ) ;
#7416=FACE_OUTER_BOUND ( 'NONE', #7054, .T. ) ;
#7434=CARTESIAN_POINT ( 'NONE',  ( 0.000000000000000000, 0.000000000000000000, 0.000000000000000000 ) ) ;
#7439=( NAMED_UNIT ( * ) PLANE_ANGLE_UNIT ( ) SI_UNIT ( $, .RADIAN. ) );
#7450=ORIENTED_EDGE ( 'NONE', *, *, #3420, .F. ) ;
#7462=ORIENTED_EDGE ( 'NONE', *, *, #6794, .F. ) ;
#7478=DIRECTION ( 'NONE',  ( 0.000000000000000000, 0.000000000000000000, 1.000000000000000000 ) ) ;
#7485=DIRECTION ( 'NONE',  ( -7.703719777548943412E-34, 0.000000000000000000, 1.000000000000000000 ) ) ;
#7534=VERTEX_POINT ( 'NONE', #942 ) ;
#7543=FACE_OUTER_BOUND ( 'NONE', #3079, .T. ) ;
#7545=AXIS2_PLACEMENT_3D ( 'NONE', #7693, #8352, #4465 ) ;
#7563=AXIS2_PLACEMENT_3D ( 'NONE', #4203, #7478, #3512 ) ;
#7568=CARTESIAN_POINT ( 'NONE',  ( 0.000000000000000000, -29.14213562373091548, -20.00000000000001776 ) ) ;
#7581=CARTESIAN_POINT ( 'NONE',  ( -5.499999999999880096, -14.99999999999990052, 79.99999999999995737 ) ) ;
#7592=ORIENTED_EDGE ( 'NONE', *, *, #5789, .F. ) ;
#7614=FACE_OUTER_BOUND ( 'NONE', #7200, .T. ) ;
#7624=EDGE_LOOP ( 'NONE', ( #3152, #6210 ) ) ;
#7630=ORIENTED_EDGE ( 'NONE', *, *, #6612, .T. ) ;
#7639=CARTESIAN_POINT ( 'NONE',  ( 2.220446049250313081E-13, -0.8578643762688908936, -20.00000000000001776 ) ) ;
#7644=( NAMED_UNIT ( * ) SI_UNIT ( $, .STERADIAN. ) SOLID_ANGLE_UNIT ( ) );
#7653=DIRECTION ( 'NONE',  ( 7.703719777548943412E-34, -0.000000000000000000, -1.000000000000000000 ) ) ;
#7693=CARTESIAN_POINT ( 'NONE',  ( 9.999999999999896971, 0.000000000000000000, 0.000000000000000000 ) ) ;
#7705=LINE ( 'NONE', #441, #6129 ) ;
#7725=EDGE_CURVE ( 'NONE', #7534, #530, #6729, .T. ) ;
#7729=CARTESIAN_POINT ( 'NONE',  ( 9.999999999999896971, 0.000000000000000000, 0.000000000000000000 ) ) ;
#7753=DIRECTION ( 'NONE',  ( -1.540743955509788682E-33, -4.592425496802573602E-17, 1.000000000000000000 ) ) ;
#7783=VECTOR ( 'NONE', #1393, 1000.000000000000000 ) ;
#7821=DIRECTION ( 'NONE',  ( 2.842664852890546338E-35, -1.000000000000000000, 0.000000000000000000 ) ) ;
#7883=VECTOR ( 'NONE', #8594, 1000.000000000000000 ) ;
#7908=VERTEX_POINT ( 'NONE', #182 ) ;
#7935=CARTESIAN_POINT ( 'NONE',  ( 0.000000000000000000, -29.14213562373091548, -1.110223024625156540E-13 ) ) ;
#7936=EDGE_CURVE ( 'NONE', #6954, #4437, #6148, .T. ) ;
#7938=CARTESIAN_POINT ( 'NONE',  ( -9.999999999999884537, -14.99999999999990052, 79.99999999999995737 ) ) ;
#7940=DIRECTION ( 'NONE',  ( 7.703719777548943412E-34, 0.000000000000000000, -1.000000000000000000 ) ) ;
#7970=DIRECTION ( 'NONE',  ( 1.000000000000000000, 0.000000000000000000, 0.000000000000000000 ) ) ;
#8000=LINE ( 'NONE', #7301, #5193 ) ;
#8030=EDGE_CURVE ( 'NONE', #5152, #4437, #5827, .T. ) ;
#8061=CIRCLE ( 'NONE', #8193, 15.00000000000000355 ) ;
#8082=ORIENTED_EDGE ( 'NONE', *, *, #5859, .T. ) ;
#8083=DIRECTION ( 'NONE',  ( 1.540743955509788682E-33, 4.592425496802573602E-17, -1.000000000000000000 ) ) ;
#8094=VERTEX_POINT ( 'NONE', #313 ) ;
#8103=AXIS2_PLACEMENT_3D ( 'NONE', #1552, #6838, #5676 ) ;
#8115=VECTOR ( 'NONE', #7485, 1000.000000000000000 ) ;
#8135=( NAMED_UNIT ( * ) SI_UNIT ( $, .STERADIAN. ) SOLID_ANGLE_UNIT ( ) );
#8150=VERTEX_POINT ( 'NONE', #1061 ) ;
#8192=EDGE_CURVE ( 'NONE', #6699, #8150, #3478, .T. ) ;
#8193=AXIS2_PLACEMENT_3D ( 'NONE', #4335, #499, #6461 ) ;
#8195=CYLINDRICAL_SURFACE ( 'NONE', #4453, 15.00000000000000355 ) ;
#8221=ORIENTED_EDGE ( 'NONE', *, *, #5752, .T. ) ;
#8226=CARTESIAN_POINT ( 'NONE',  ( 9.999999999999896971, 0.000000000000000000, 0.000000000000000000 ) ) ;
#8237=DIRECTION ( 'NONE',  ( 1.000000000000000000, 0.000000000000000000, 0.000000000000000000 ) ) ;
#8251=FACE_OUTER_BOUND ( 'NONE', #2837, .T. ) ;
#8254=FACE_OUTER_BOUND ( 'NONE', #3790, .T. ) ;
#8256=DIRECTION ( 'NONE',  ( -7.703719777548943412E-34, 0.000000000000000000, 1.000000000000000000 ) ) ;
#8310=DIRECTION ( 'NONE',  ( 1.000000000000000000, 0.000000000000000000, 0.000000000000000000 ) ) ;
#8352=DIRECTION ( 'NONE',  ( -1.000000000000000000, 2.842664852890546338E-35, -7.703719777548943412E-34 ) ) ;
#8385=CARTESIAN_POINT ( 'NONE',  ( -2.220446049250313081E-13, -650.0000000000000000, 79.99999999999995737 ) ) ;
#8416=LINE ( 'NONE', #2440, #3375 ) ;
#8418=VERTEX_POINT ( 'NONE', #3078 ) ;
#8434=DIRECTION ( 'NONE',  ( -7.703719777548943412E-34, 0.000000000000000000, 1.000000000000000000 ) ) ;
#8469=DIRECTION ( 'NONE',  ( -7.703719777548943412E-34, 0.000000000000000000, 1.000000000000000000 ) ) ;
#8486=ORIENTED_EDGE ( 'NONE', *, *, #6627, .F. ) ;
#8488=DIRECTION ( 'NONE',  ( -7.703719777548943412E-34, 0.000000000000000000, 1.000000000000000000 ) ) ;
#8491=ORIENTED_EDGE ( 'NONE', *, *, #5062, .F. ) ;
#8564=ORIENTED_EDGE ( 'NONE', *, *, #8192, .T. ) ;
#8584=ORIENTED_EDGE ( 'NONE', *, *, #6341, .F. ) ;
#8594=DIRECTION ( 'NONE',  ( -1.000000000000000000, 2.842664852890546338E-35, 1.540743955509788340E-33 ) ) ;
#8671=COLOUR_RGB('Off White',0.89,0.88,0.83);
#8672=FILL_AREA_STYLE_COLOUR('',#8671);
#8673=FILL_AREA_STYLE('',(#8672));
#8674=SURFACE_STYLE_FILL_AREA(#8673);
#8675=SURFACE_SIDE_STYLE('',(#8674));
#8676=SURFACE_STYLE_USAGE(.BOTH.,#8675);
#8677=PRESENTATION_STYLE_ASSIGNMENT((#8676));
ENDSEC;
END-ISO-10303-21;
